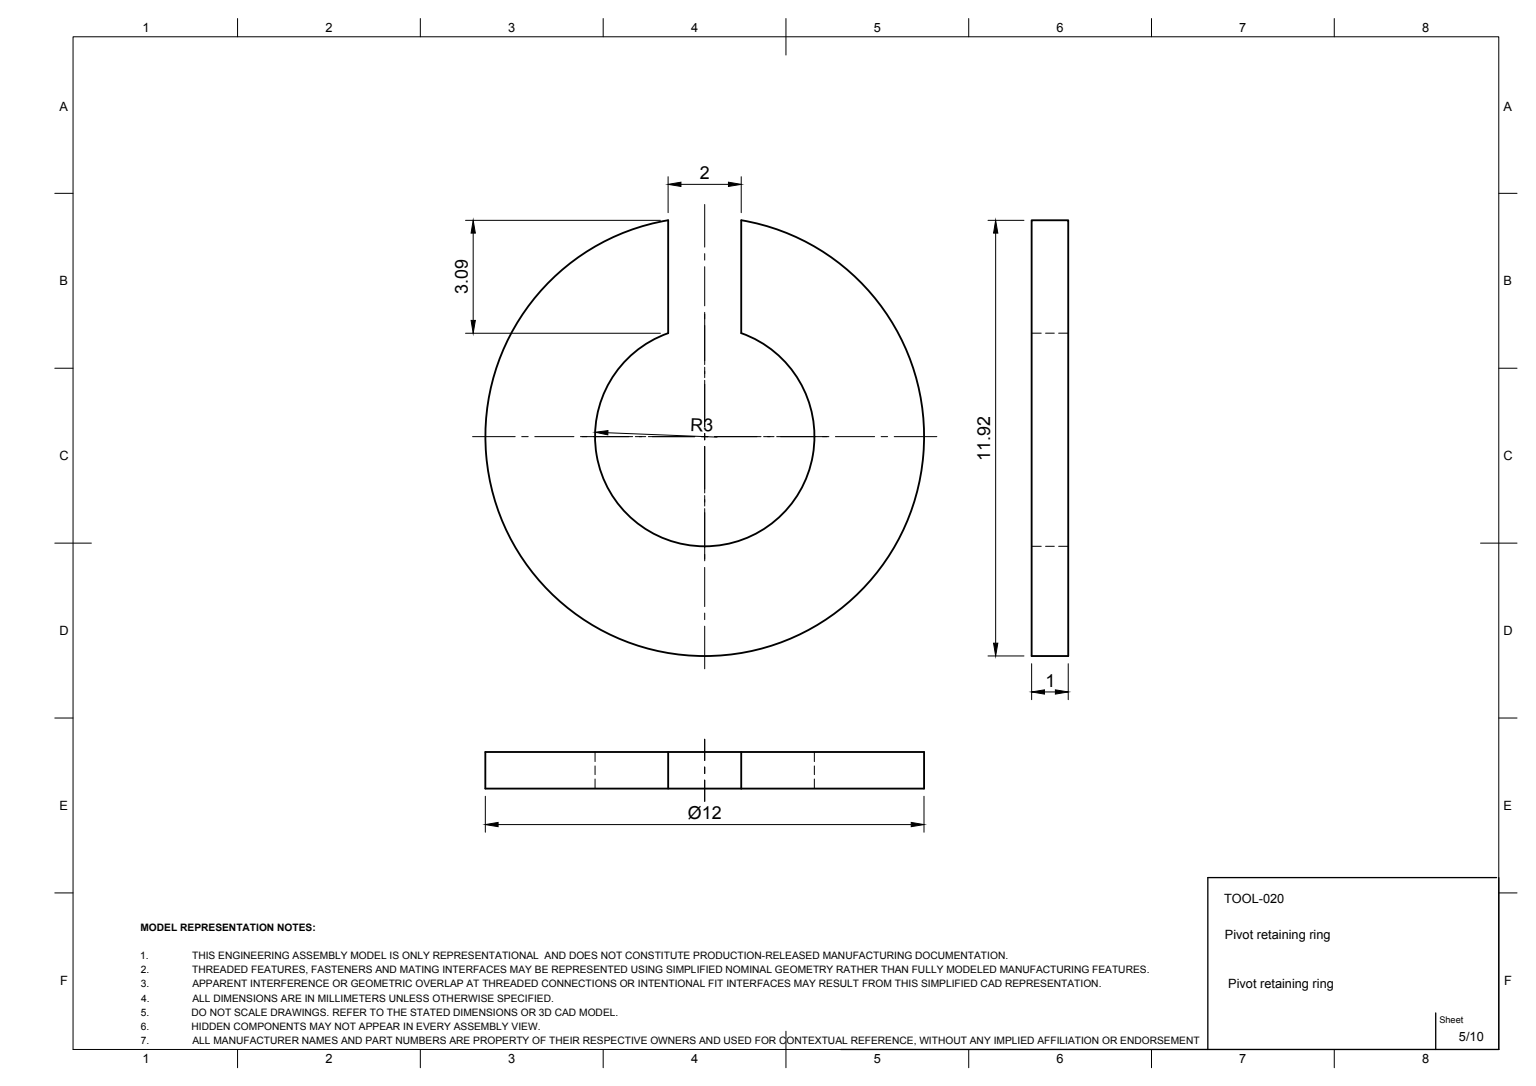
ISO-10303-21;
HEADER;
/* Generated by software containing ST-Developer
 * from STEP Tools, Inc. (www.steptools.com) 
 */

FILE_DESCRIPTION(
/* description */ (''),
/* implementation_level */ '2;1');

FILE_NAME(
/* name */ 'Pivot retaining ring.step',
/* time_stamp */ '2026-11-10T09:09:39-08:00',
/* author */ (''),
/* organization */ (''),
/* preprocessor_version */ 'ST-DEVELOPER v20.2',
/* originating_system */ 'Autodesk Translation Framework v15.17.0.0',
/* authorisation */ '');

FILE_SCHEMA (('AUTOMOTIVE_DESIGN { 1 0 10303 214 3 1 1 }'));
ENDSEC;

DATA;
#10=MECHANICAL_DESIGN_GEOMETRIC_PRESENTATION_REPRESENTATION('',(#557),#18353);
#539=SHAPE_REPRESENTATION_RELATIONSHIP('SRR','None',#18399,#548);
#548=ADVANCED_BREP_SHAPE_REPRESENTATION('',(#566),#18345);
#557=STYLED_ITEM('',(#18458),#566);
#566=MANIFOLD_SOLID_BREP('Body1',#6488);
#664=PLANE('',#6675);
#665=PLANE('',#6676);
#666=PLANE('',#6677);
#667=PLANE('',#6684);
#823=FACE_OUTER_BOUND('',#1207,.T.);
#824=FACE_OUTER_BOUND('',#1208,.T.);
#825=FACE_OUTER_BOUND('',#1209,.T.);
#826=FACE_OUTER_BOUND('',#1210,.T.);
#827=FACE_OUTER_BOUND('',#1211,.T.);
#828=FACE_OUTER_BOUND('',#1212,.T.);
#1207=EDGE_LOOP('',(#4306,#4307,#4308,#4309));
#1208=EDGE_LOOP('',(#4310,#4311,#4312,#4313));
#1209=EDGE_LOOP('',(#4314,#4315,#4316,#4317));
#1210=EDGE_LOOP('',(#4318,#4319,#4320,#4321));
#1211=EDGE_LOOP('',(#4322,#4323,#4324,#4325));
#1212=EDGE_LOOP('',(#4326,#4327,#4328,#4329));
#1655=LINE('',#8672,#2059);
#1656=LINE('',#8674,#2060);
#1657=LINE('',#8676,#2061);
#1658=LINE('',#8677,#2062);
#1659=LINE('',#8681,#2063);
#1660=LINE('',#8683,#2064);
#1661=LINE('',#8685,#2065);
#1662=LINE('',#8686,#2066);
#2059=VECTOR('',#7308,1.);
#2060=VECTOR('',#7309,1.);
#2061=VECTOR('',#7310,1.);
#2062=VECTOR('',#7311,1.);
#2063=VECTOR('',#7314,1.);
#2064=VECTOR('',#7315,1.);
#2065=VECTOR('',#7316,1.);
#2066=VECTOR('',#7317,1.);
#2434=CIRCLE('',#6678,0.6);
#2435=CIRCLE('',#6679,0.3);
#2436=CIRCLE('',#6681,0.3);
#2437=CIRCLE('',#6683,0.6);
#2631=VERTEX_POINT('',#8670);
#2632=VERTEX_POINT('',#8671);
#2633=VERTEX_POINT('',#8673);
#2634=VERTEX_POINT('',#8675);
#2635=VERTEX_POINT('',#8679);
#2636=VERTEX_POINT('',#8680);
#2637=VERTEX_POINT('',#8682);
#2638=VERTEX_POINT('',#8684);
#3270=EDGE_CURVE('',#2631,#2632,#1655,.T.);
#3271=EDGE_CURVE('',#2633,#2631,#1656,.T.);
#3272=EDGE_CURVE('',#2634,#2633,#1657,.T.);
#3273=EDGE_CURVE('',#2632,#2634,#1658,.T.);
#3274=EDGE_CURVE('',#2635,#2636,#1659,.T.);
#3275=EDGE_CURVE('',#2637,#2635,#1660,.T.);
#3276=EDGE_CURVE('',#2638,#2637,#1661,.T.);
#3277=EDGE_CURVE('',#2636,#2638,#1662,.T.);
#3278=EDGE_CURVE('',#2633,#2638,#2434,.T.);
#3279=EDGE_CURVE('',#2636,#2631,#2435,.T.);
#3280=EDGE_CURVE('',#2635,#2632,#2436,.T.);
#3281=EDGE_CURVE('',#2634,#2637,#2437,.T.);
#4306=ORIENTED_EDGE('',*,*,#3270,.F.);
#4307=ORIENTED_EDGE('',*,*,#3271,.F.);
#4308=ORIENTED_EDGE('',*,*,#3272,.F.);
#4309=ORIENTED_EDGE('',*,*,#3273,.F.);
#4310=ORIENTED_EDGE('',*,*,#3274,.F.);
#4311=ORIENTED_EDGE('',*,*,#3275,.F.);
#4312=ORIENTED_EDGE('',*,*,#3276,.F.);
#4313=ORIENTED_EDGE('',*,*,#3277,.F.);
#4314=ORIENTED_EDGE('',*,*,#3277,.T.);
#4315=ORIENTED_EDGE('',*,*,#3278,.F.);
#4316=ORIENTED_EDGE('',*,*,#3271,.T.);
#4317=ORIENTED_EDGE('',*,*,#3279,.F.);
#4318=ORIENTED_EDGE('',*,*,#3274,.T.);
#4319=ORIENTED_EDGE('',*,*,#3279,.T.);
#4320=ORIENTED_EDGE('',*,*,#3270,.T.);
#4321=ORIENTED_EDGE('',*,*,#3280,.F.);
#4322=ORIENTED_EDGE('',*,*,#3276,.T.);
#4323=ORIENTED_EDGE('',*,*,#3281,.F.);
#4324=ORIENTED_EDGE('',*,*,#3272,.T.);
#4325=ORIENTED_EDGE('',*,*,#3278,.T.);
#4326=ORIENTED_EDGE('',*,*,#3275,.T.);
#4327=ORIENTED_EDGE('',*,*,#3280,.T.);
#4328=ORIENTED_EDGE('',*,*,#3273,.T.);
#4329=ORIENTED_EDGE('',*,*,#3281,.T.);
#5996=CYLINDRICAL_SURFACE('',#6680,0.3);
#5997=CYLINDRICAL_SURFACE('',#6682,0.6);
#6154=ADVANCED_FACE('',(#823),#664,.F.);
#6155=ADVANCED_FACE('',(#824),#665,.F.);
#6156=ADVANCED_FACE('',(#825),#666,.F.);
#6157=ADVANCED_FACE('',(#826),#5996,.F.);
#6158=ADVANCED_FACE('',(#827),#5997,.T.);
#6159=ADVANCED_FACE('',(#828),#667,.T.);
#6488=CLOSED_SHELL('',(#6154,#6155,#6156,#6157,#6158,#6159));
#6674=AXIS2_PLACEMENT_3D('',#8668,#7304,#7305);
#6675=AXIS2_PLACEMENT_3D('',#8669,#7306,#7307);
#6676=AXIS2_PLACEMENT_3D('',#8678,#7312,#7313);
#6677=AXIS2_PLACEMENT_3D('',#8687,#7318,#7319);
#6678=AXIS2_PLACEMENT_3D('',#8688,#7320,#7321);
#6679=AXIS2_PLACEMENT_3D('',#8689,#7322,#7323);
#6680=AXIS2_PLACEMENT_3D('',#8690,#7324,#7325);
#6681=AXIS2_PLACEMENT_3D('',#8691,#7326,#7327);
#6682=AXIS2_PLACEMENT_3D('',#8692,#7328,#7329);
#6683=AXIS2_PLACEMENT_3D('',#8693,#7330,#7331);
#6684=AXIS2_PLACEMENT_3D('',#8694,#7332,#7333);
#7304=DIRECTION('axis',(0.,0.,1.));
#7305=DIRECTION('refdir',(1.,0.,0.));
#7306=DIRECTION('center_axis',(-1.,0.,0.));
#7307=DIRECTION('ref_axis',(0.,1.,0.));
#7308=DIRECTION('',(0.,0.,1.));
#7309=DIRECTION('',(0.,-1.,0.));
#7310=DIRECTION('',(0.,0.,-1.));
#7311=DIRECTION('',(0.,1.,0.));
#7312=DIRECTION('center_axis',(1.,0.,0.));
#7313=DIRECTION('ref_axis',(0.,-1.,0.));
#7314=DIRECTION('',(0.,0.,-1.));
#7315=DIRECTION('',(0.,-1.,0.));
#7316=DIRECTION('',(0.,0.,1.));
#7317=DIRECTION('',(0.,1.,0.));
#7318=DIRECTION('center_axis',(0.,0.,1.));
#7319=DIRECTION('ref_axis',(1.,0.,0.));
#7320=DIRECTION('center_axis',(0.,0.,1.));
#7321=DIRECTION('ref_axis',(1.,0.,0.));
#7322=DIRECTION('center_axis',(0.,0.,-1.));
#7323=DIRECTION('ref_axis',(1.,0.,0.));
#7324=DIRECTION('center_axis',(0.,0.,1.));
#7325=DIRECTION('ref_axis',(6.12323399573677E-17,-1.,0.));
#7326=DIRECTION('center_axis',(0.,0.,-1.));
#7327=DIRECTION('ref_axis',(1.,0.,0.));
#7328=DIRECTION('center_axis',(0.,0.,1.));
#7329=DIRECTION('ref_axis',(6.12323399573677E-17,-1.,0.));
#7330=DIRECTION('center_axis',(0.,0.,1.));
#7331=DIRECTION('ref_axis',(1.,0.,0.));
#7332=DIRECTION('center_axis',(0.,0.,1.));
#7333=DIRECTION('ref_axis',(1.,0.,0.));
#8668=CARTESIAN_POINT('',(0.,0.,0.));
#8669=CARTESIAN_POINT('Origin',(-0.1,0.,0.1));
#8670=CARTESIAN_POINT('',(-0.1,0.282842712474619,0.));
#8671=CARTESIAN_POINT('',(-0.1,0.282842712474619,0.1));
#8672=CARTESIAN_POINT('',(-0.1,0.282842712474619,0.));
#8673=CARTESIAN_POINT('',(-0.1,0.591607978309962,0.));
#8674=CARTESIAN_POINT('',(-0.1,0.,0.));
#8675=CARTESIAN_POINT('',(-0.1,0.591607978309962,0.1));
#8676=CARTESIAN_POINT('',(-0.1,0.591607978309962,0.));
#8677=CARTESIAN_POINT('',(-0.1,0.,0.1));
#8678=CARTESIAN_POINT('Origin',(0.1,1.2,0.1));
#8679=CARTESIAN_POINT('',(0.1,0.282842712474619,0.1));
#8680=CARTESIAN_POINT('',(0.1,0.282842712474619,0.));
#8681=CARTESIAN_POINT('',(0.1,0.282842712474619,0.));
#8682=CARTESIAN_POINT('',(0.1,0.591607978309962,0.1));
#8683=CARTESIAN_POINT('',(0.1,0.6,0.1));
#8684=CARTESIAN_POINT('',(0.1,0.591607978309962,0.));
#8685=CARTESIAN_POINT('',(0.1,0.591607978309962,0.));
#8686=CARTESIAN_POINT('',(0.1,0.6,0.));
#8687=CARTESIAN_POINT('Origin',(0.,0.,0.));
#8688=CARTESIAN_POINT('Origin',(0.,0.,0.));
#8689=CARTESIAN_POINT('Origin',(0.,0.,0.));
#8690=CARTESIAN_POINT('Origin',(0.,0.,0.));
#8691=CARTESIAN_POINT('Origin',(0.,0.,0.1));
#8692=CARTESIAN_POINT('Origin',(0.,0.,0.));
#8693=CARTESIAN_POINT('Origin',(0.,0.,0.1));
#8694=CARTESIAN_POINT('Origin',(0.,0.,0.1));
#18333=UNCERTAINTY_MEASURE_WITH_UNIT(LENGTH_MEASURE(0.001),#18354,
'DISTANCE_ACCURACY_VALUE',
'Maximum model space distance between geometric entities at asserted c
onnectivities');
#18341=UNCERTAINTY_MEASURE_WITH_UNIT(LENGTH_MEASURE(0.001),#18354,
'DISTANCE_ACCURACY_VALUE',
'Maximum model space distance between geometric entities at asserted c
onnectivities');
#18345=(
GEOMETRIC_REPRESENTATION_CONTEXT(3)
GLOBAL_UNCERTAINTY_ASSIGNED_CONTEXT((#18333))
GLOBAL_UNIT_ASSIGNED_CONTEXT((#18354,#18356,#18357))
REPRESENTATION_CONTEXT('','3D')
);
#18353=(
GEOMETRIC_REPRESENTATION_CONTEXT(3)
GLOBAL_UNCERTAINTY_ASSIGNED_CONTEXT((#18341))
GLOBAL_UNIT_ASSIGNED_CONTEXT((#18354,#18356,#18357))
REPRESENTATION_CONTEXT('','3D')
);
#18354=(
LENGTH_UNIT()
NAMED_UNIT(*)
SI_UNIT(.CENTI.,.METRE.)
);
#18356=(
NAMED_UNIT(*)
PLANE_ANGLE_UNIT()
SI_UNIT($,.RADIAN.)
);
#18357=(
NAMED_UNIT(*)
SI_UNIT($,.STERADIAN.)
SOLID_ANGLE_UNIT()
);
#18361=SHAPE_DEFINITION_REPRESENTATION(#18372,#18399);
#18372=PRODUCT_DEFINITION_SHAPE('',$,#18411);
#18399=SHAPE_REPRESENTATION('',(#6674),#18345);
#18407=PRODUCT_DEFINITION_CONTEXT('part definition',#18442,'design');
#18411=PRODUCT_DEFINITION('Pivot retaining ring','Pivot retaining ring',
#18422,#18407);
#18422=PRODUCT_DEFINITION_FORMATION('',$,#18447);
#18442=APPLICATION_CONTEXT(
'Core Data for Automotive Mechanical Design Process');
#18443=PRODUCT_CONTEXT('part definition',#18442,'mechanical');
#18447=PRODUCT('Pivot retaining ring','Pivot retaining ring',$,(#18443));
#18458=PRESENTATION_STYLE_ASSIGNMENT((#18466));
#18466=SURFACE_STYLE_USAGE(.BOTH.,#18474);
#18474=SURFACE_SIDE_STYLE('',(#18482));
#18482=SURFACE_STYLE_FILL_AREA(#18490);
#18490=FILL_AREA_STYLE('Dark gray',(#18498));
#18498=FILL_AREA_STYLE_COLOUR('Dark gray',#18506);
#18506=COLOUR_RGB('Dark gray',0.250980392156863,0.282352941176471,0.32156862745098);
ENDSEC;
END-ISO-10303-21;
